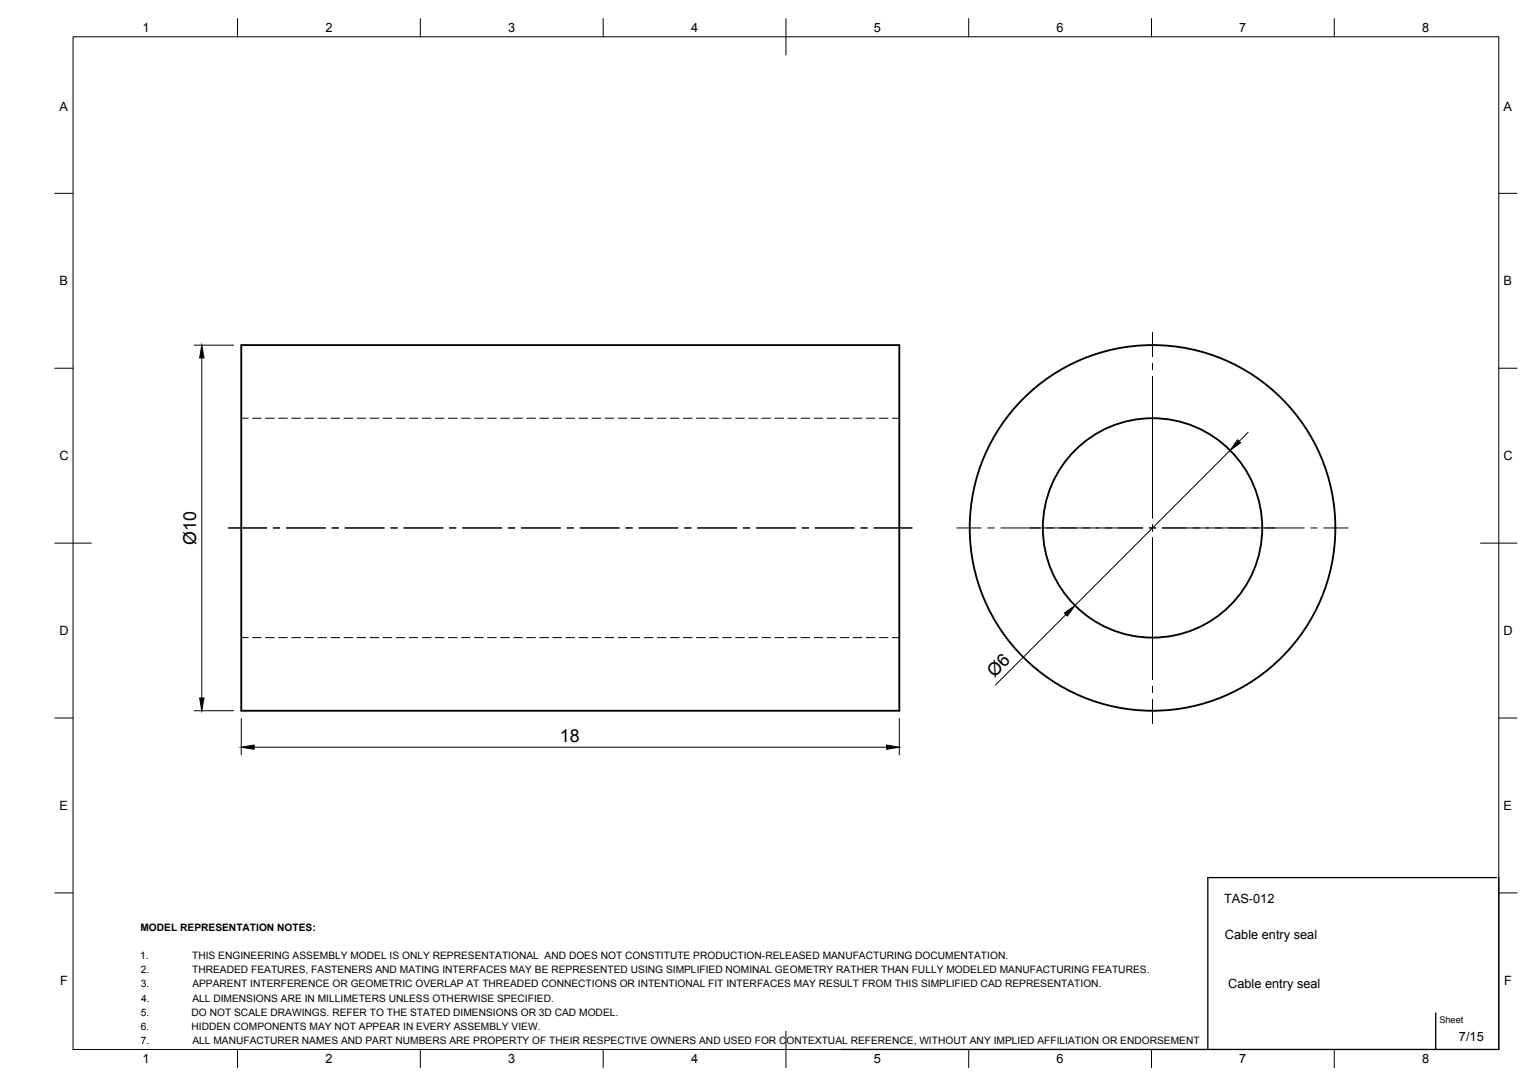
ISO-10303-21;
HEADER;
/* Generated by software containing ST-Developer
 * from STEP Tools, Inc. (www.steptools.com) 
 */

FILE_DESCRIPTION(
/* description */ (
'Independent welded steel electronics enclosure with removable sealed 
lid, internal mounting tray and two threaded cable entries. 300 x 220 
mm body. No ingress or electrical safety rating assigned.'),
/* implementation_level */ '2;1');

FILE_NAME(
/* name */ 'Cable entry seal.step',
/* time_stamp */ '2026-11-14T09:13:27-08:00',
/* author */ (''),
/* organization */ (''),
/* preprocessor_version */ 'ST-DEVELOPER v20.2',
/* originating_system */ 'Autodesk Translation Framework v15.17.0.0',
/* authorisation */ '');

FILE_SCHEMA (('AUTOMOTIVE_DESIGN { 1 0 10303 214 3 1 1 }'));
ENDSEC;

DATA;
#10=MECHANICAL_DESIGN_GEOMETRIC_PRESENTATION_REPRESENTATION('',(#980),#94412);
#950=SHAPE_REPRESENTATION_RELATIONSHIP('SRR','None',#94502,#965);
#965=ADVANCED_BREP_SHAPE_REPRESENTATION('',(#995),#94411);
#980=STYLED_ITEM('',(#94578),#995);
#995=MANIFOLD_SOLID_BREP('Body1',#8265);
#1056=FACE_BOUND('',#1929,.T.);
#1057=FACE_BOUND('',#1931,.T.);
#1156=PLANE('',#8922);
#1157=PLANE('',#8923);
#1510=FACE_OUTER_BOUND('',#1926,.T.);
#1511=FACE_OUTER_BOUND('',#1927,.T.);
#1512=FACE_OUTER_BOUND('',#1928,.T.);
#1513=FACE_OUTER_BOUND('',#1930,.T.);
#1926=EDGE_LOOP('',(#7646,#7647,#7648,#7649));
#1927=EDGE_LOOP('',(#7650,#7651,#7652,#7653));
#1928=EDGE_LOOP('',(#7654));
#1929=EDGE_LOOP('',(#7655));
#1930=EDGE_LOOP('',(#7656));
#1931=EDGE_LOOP('',(#7657));
#2328=LINE('',#94349,#2726);
#2329=LINE('',#94355,#2727);
#2726=VECTOR('',#10310,3.);
#2727=VECTOR('',#10317,5.);
#2842=CIRCLE('',#8917,3.);
#2843=CIRCLE('',#8918,3.);
#2844=CIRCLE('',#8920,5.);
#2845=CIRCLE('',#8921,5.);
#3808=VERTEX_POINT('',#94346);
#3809=VERTEX_POINT('',#94348);
#3810=VERTEX_POINT('',#94352);
#3811=VERTEX_POINT('',#94354);
#5088=EDGE_CURVE('',#3808,#3808,#2842,.T.);
#5089=EDGE_CURVE('',#3808,#3809,#2328,.T.);
#5090=EDGE_CURVE('',#3809,#3809,#2843,.T.);
#5091=EDGE_CURVE('',#3810,#3810,#2844,.T.);
#5092=EDGE_CURVE('',#3810,#3811,#2329,.T.);
#5093=EDGE_CURVE('',#3811,#3811,#2845,.T.);
#7646=ORIENTED_EDGE('',*,*,#5088,.T.);
#7647=ORIENTED_EDGE('',*,*,#5089,.T.);
#7648=ORIENTED_EDGE('',*,*,#5090,.F.);
#7649=ORIENTED_EDGE('',*,*,#5089,.F.);
#7650=ORIENTED_EDGE('',*,*,#5091,.F.);
#7651=ORIENTED_EDGE('',*,*,#5092,.T.);
#7652=ORIENTED_EDGE('',*,*,#5093,.T.);
#7653=ORIENTED_EDGE('',*,*,#5092,.F.);
#7654=ORIENTED_EDGE('',*,*,#5091,.T.);
#7655=ORIENTED_EDGE('',*,*,#5090,.T.);
#7656=ORIENTED_EDGE('',*,*,#5093,.F.);
#7657=ORIENTED_EDGE('',*,*,#5088,.F.);
#7893=CYLINDRICAL_SURFACE('',#8916,3.);
#7894=CYLINDRICAL_SURFACE('',#8919,5.);
#8247=ADVANCED_FACE('',(#1510),#7893,.F.);
#8248=ADVANCED_FACE('',(#1511),#7894,.T.);
#8249=ADVANCED_FACE('',(#1512,#1056),#1156,.T.);
#8250=ADVANCED_FACE('',(#1513,#1057),#1157,.F.);
#8265=CLOSED_SHELL('',(#8247,#8248,#8249,#8250));
#8915=AXIS2_PLACEMENT_3D('',#94344,#10304,#10305);
#8916=AXIS2_PLACEMENT_3D('',#94345,#10306,#10307);
#8917=AXIS2_PLACEMENT_3D('',#94347,#10308,#10309);
#8918=AXIS2_PLACEMENT_3D('',#94350,#10311,#10312);
#8919=AXIS2_PLACEMENT_3D('',#94351,#10313,#10314);
#8920=AXIS2_PLACEMENT_3D('',#94353,#10315,#10316);
#8921=AXIS2_PLACEMENT_3D('',#94356,#10318,#10319);
#8922=AXIS2_PLACEMENT_3D('',#94357,#10320,#10321);
#8923=AXIS2_PLACEMENT_3D('',#94358,#10322,#10323);
#10304=DIRECTION('axis',(0.,0.,1.));
#10305=DIRECTION('refdir',(1.,0.,0.));
#10306=DIRECTION('center_axis',(0.,0.,1.));
#10307=DIRECTION('ref_axis',(1.,0.,0.));
#10308=DIRECTION('center_axis',(0.,0.,-1.));
#10309=DIRECTION('ref_axis',(1.,0.,0.));
#10310=DIRECTION('',(0.,0.,1.));
#10311=DIRECTION('center_axis',(0.,0.,-1.));
#10312=DIRECTION('ref_axis',(1.,0.,0.));
#10313=DIRECTION('center_axis',(0.,0.,1.));
#10314=DIRECTION('ref_axis',(1.,0.,0.));
#10315=DIRECTION('center_axis',(0.,0.,1.));
#10316=DIRECTION('ref_axis',(1.,0.,0.));
#10317=DIRECTION('',(0.,0.,-1.));
#10318=DIRECTION('center_axis',(0.,0.,1.));
#10319=DIRECTION('ref_axis',(1.,0.,0.));
#10320=DIRECTION('center_axis',(0.,0.,1.));
#10321=DIRECTION('ref_axis',(1.,0.,0.));
#10322=DIRECTION('center_axis',(0.,0.,1.));
#10323=DIRECTION('ref_axis',(1.,0.,0.));
#94344=CARTESIAN_POINT('',(0.,0.,0.));
#94345=CARTESIAN_POINT('Origin',(0.,0.,0.));
#94346=CARTESIAN_POINT('',(-3.,-3.67394039744206E-16,0.));
#94347=CARTESIAN_POINT('Origin',(0.,0.,0.));
#94348=CARTESIAN_POINT('',(-3.,-3.67394039744206E-16,18.));
#94349=CARTESIAN_POINT('',(-3.,-3.67394039744206E-16,0.));
#94350=CARTESIAN_POINT('Origin',(0.,0.,18.));
#94351=CARTESIAN_POINT('Origin',(0.,0.,0.));
#94352=CARTESIAN_POINT('',(-5.,-6.12323399573677E-16,18.));
#94353=CARTESIAN_POINT('Origin',(0.,0.,18.));
#94354=CARTESIAN_POINT('',(-5.,-6.12323399573677E-16,0.));
#94355=CARTESIAN_POINT('',(-5.,-6.12323399573677E-16,0.));
#94356=CARTESIAN_POINT('Origin',(0.,0.,0.));
#94357=CARTESIAN_POINT('Origin',(0.,0.,18.));
#94358=CARTESIAN_POINT('Origin',(0.,0.,0.));
#94393=UNCERTAINTY_MEASURE_WITH_UNIT(LENGTH_MEASURE(0.01),#94413,
'DISTANCE_ACCURACY_VALUE',
'Maximum model space distance between geometric entities at asserted c
onnectivities');
#94394=UNCERTAINTY_MEASURE_WITH_UNIT(LENGTH_MEASURE(0.01),#94413,
'DISTANCE_ACCURACY_VALUE',
'Maximum model space distance between geometric entities at asserted c
onnectivities');
#94411=(
GEOMETRIC_REPRESENTATION_CONTEXT(3)
GLOBAL_UNCERTAINTY_ASSIGNED_CONTEXT((#94393))
GLOBAL_UNIT_ASSIGNED_CONTEXT((#94413,#94415,#94416))
REPRESENTATION_CONTEXT('','3D')
);
#94412=(
GEOMETRIC_REPRESENTATION_CONTEXT(3)
GLOBAL_UNCERTAINTY_ASSIGNED_CONTEXT((#94394))
GLOBAL_UNIT_ASSIGNED_CONTEXT((#94413,#94415,#94416))
REPRESENTATION_CONTEXT('','3D')
);
#94413=(
LENGTH_UNIT()
NAMED_UNIT(*)
SI_UNIT(.MILLI.,.METRE.)
);
#94415=(
NAMED_UNIT(*)
PLANE_ANGLE_UNIT()
SI_UNIT($,.RADIAN.)
);
#94416=(
NAMED_UNIT(*)
SI_UNIT($,.STERADIAN.)
SOLID_ANGLE_UNIT()
);
#94433=SHAPE_DEFINITION_REPRESENTATION(#94467,#94502);
#94467=PRODUCT_DEFINITION_SHAPE('',$,#94520);
#94502=SHAPE_REPRESENTATION('',(#8915),#94411);
#94503=PRODUCT_DEFINITION_CONTEXT('part definition',#94556,'design');
#94520=PRODUCT_DEFINITION('Cable entry seal','Cable entry seal',#94537,
#94503);
#94537=PRODUCT_DEFINITION_FORMATION('',$,#94574);
#94556=APPLICATION_CONTEXT(
'Core Data for Automotive Mechanical Design Process');
#94557=PRODUCT_CONTEXT('part definition',#94556,'mechanical');
#94574=PRODUCT('Cable entry seal','Cable entry seal',$,(#94557));
#94578=PRESENTATION_STYLE_ASSIGNMENT((#94585));
#94585=SURFACE_STYLE_USAGE(.BOTH.,#94592);
#94592=SURFACE_SIDE_STYLE('',(#94599));
#94599=SURFACE_STYLE_FILL_AREA(#94606);
#94606=FILL_AREA_STYLE('Opaque(64,72,82)',(#94613));
#94613=FILL_AREA_STYLE_COLOUR('Opaque(64,72,82)',#94620);
#94620=COLOUR_RGB('Opaque(64,72,82)',0.250980392156863,0.282352941176471,
0.32156862745098);
ENDSEC;
END-ISO-10303-21;
